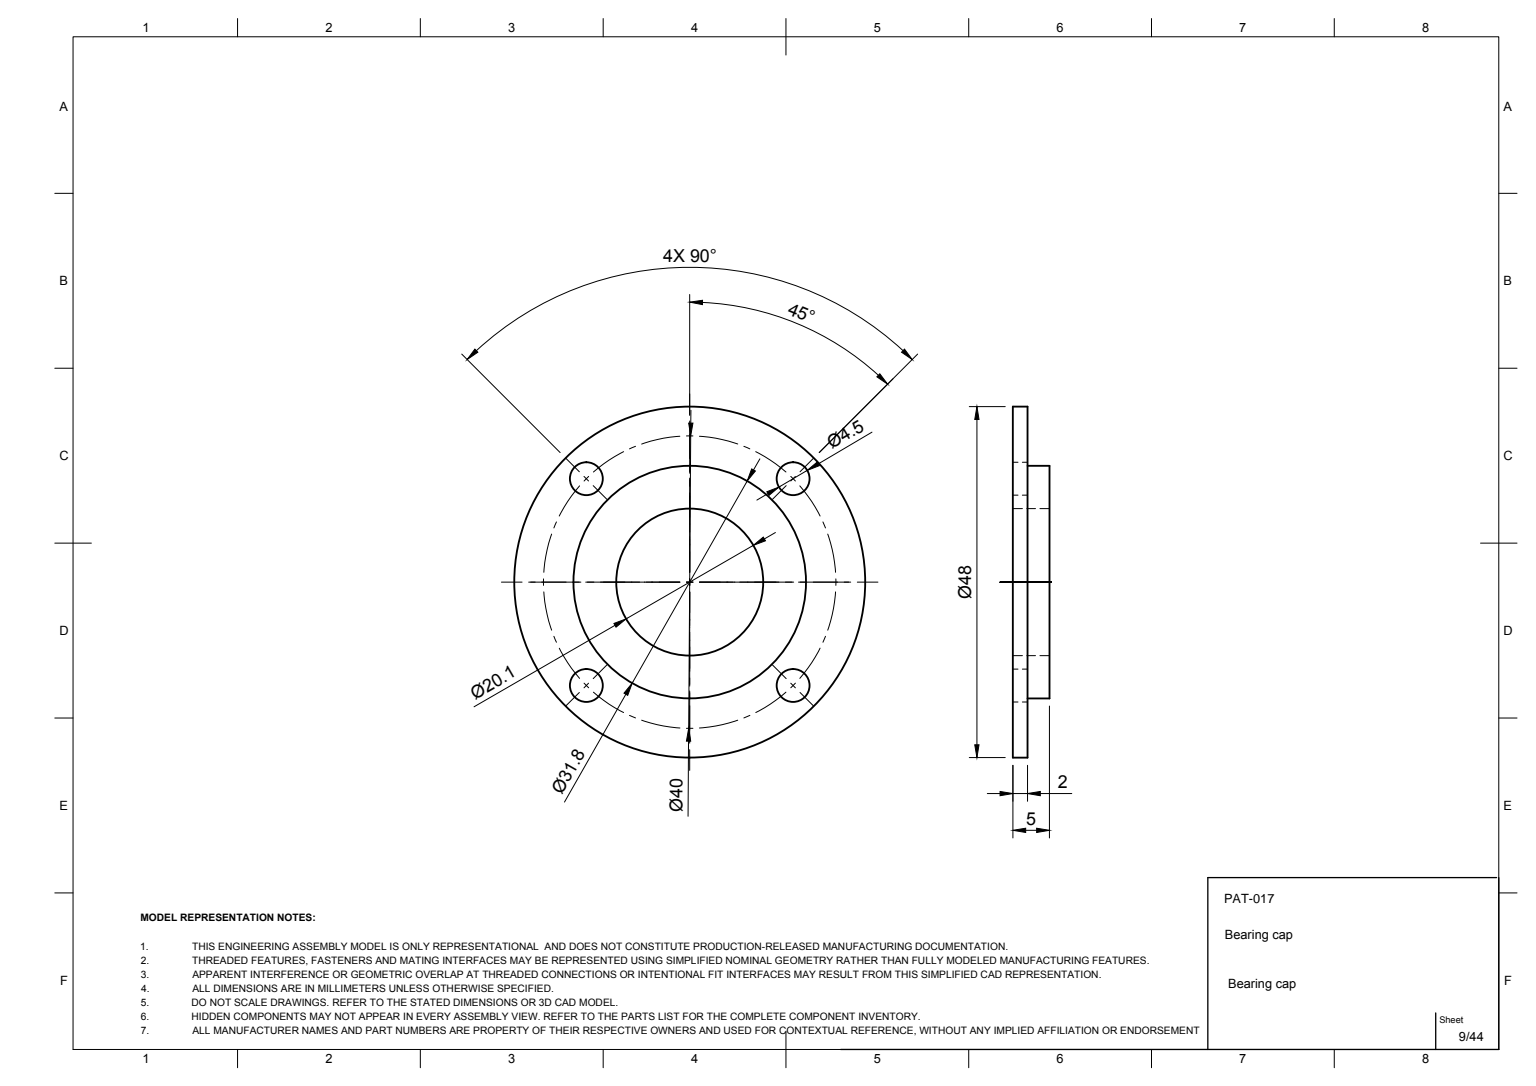
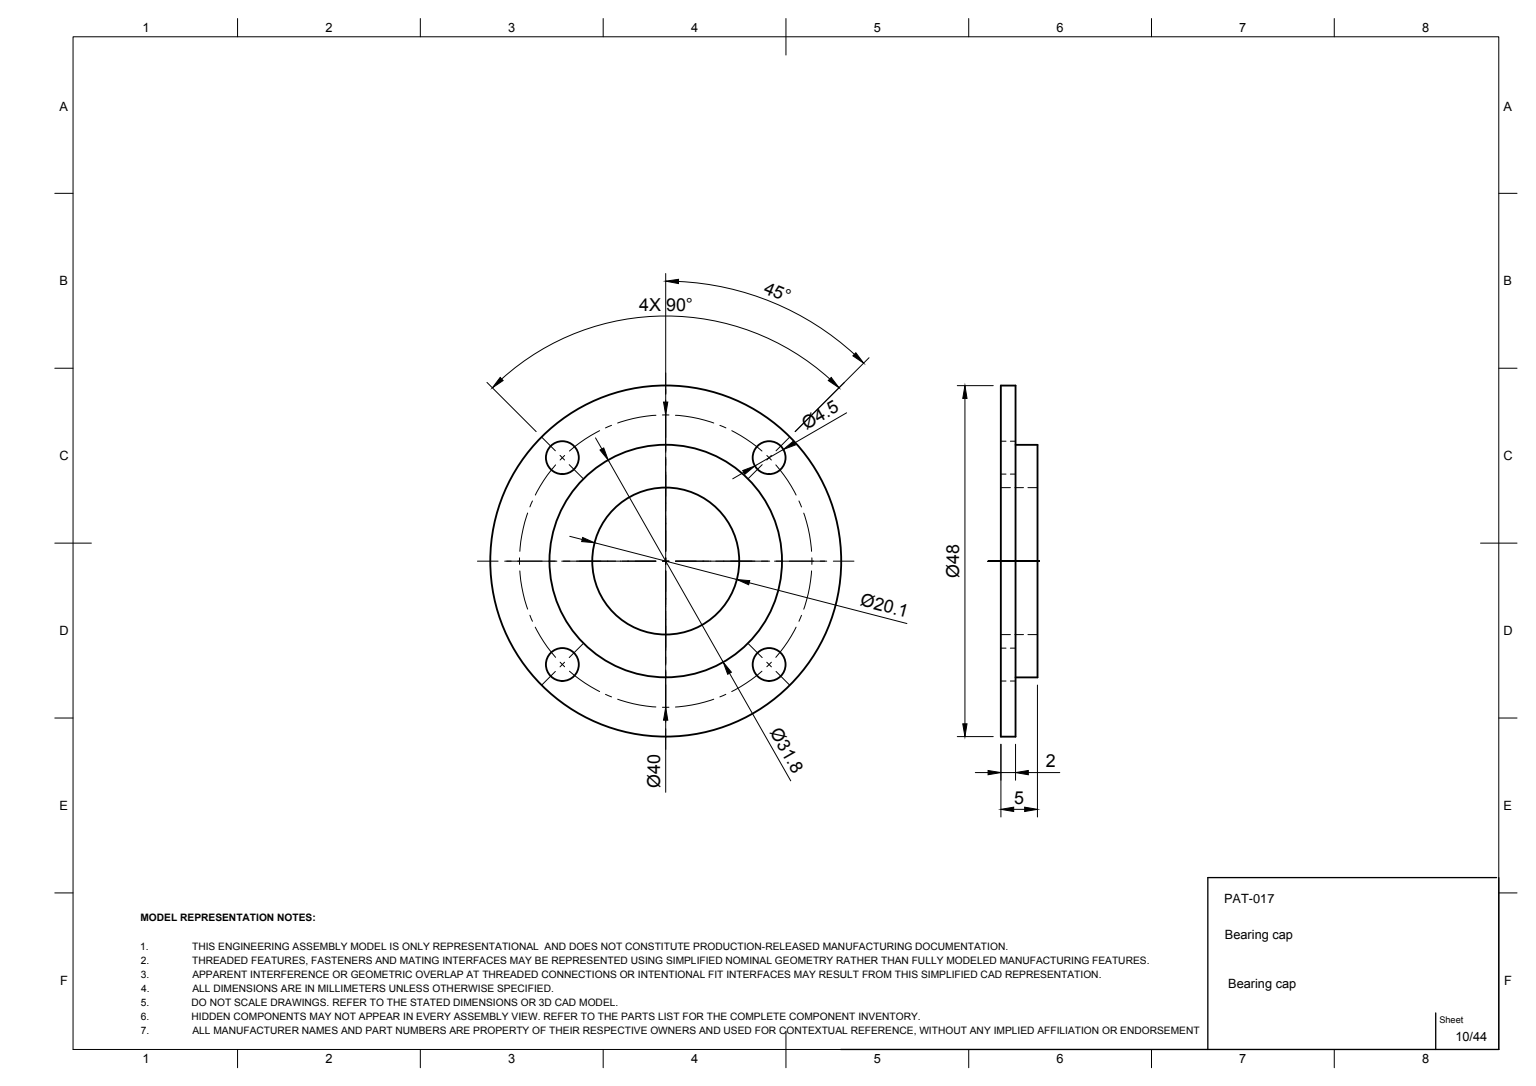
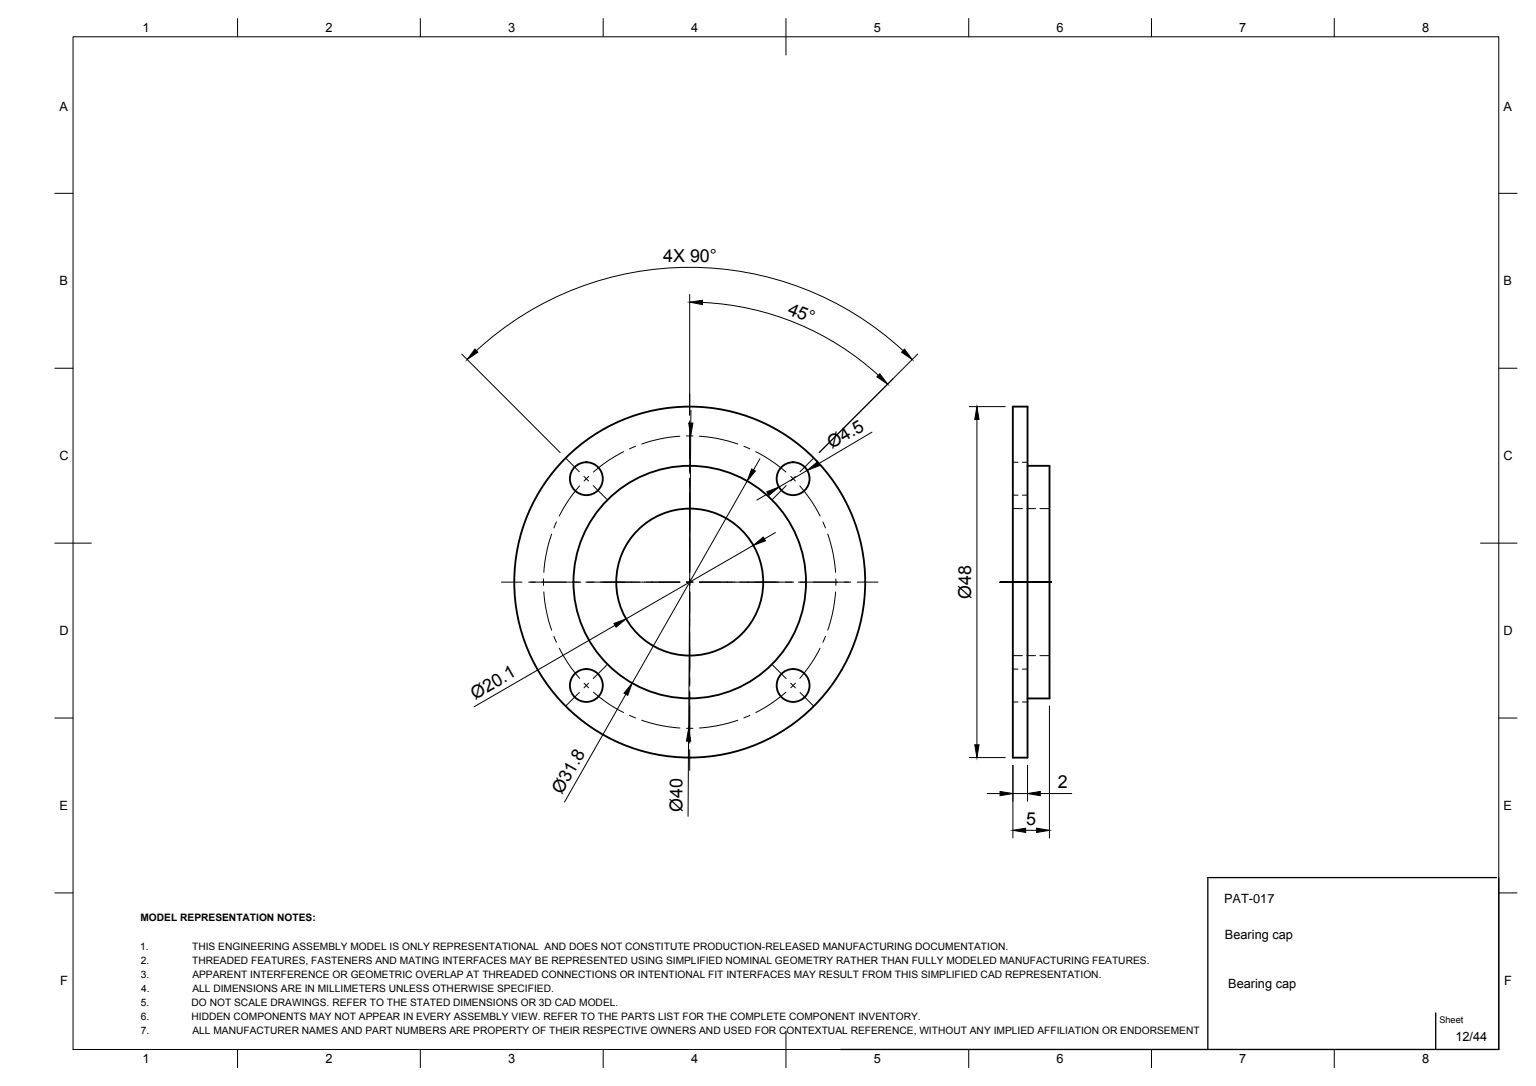
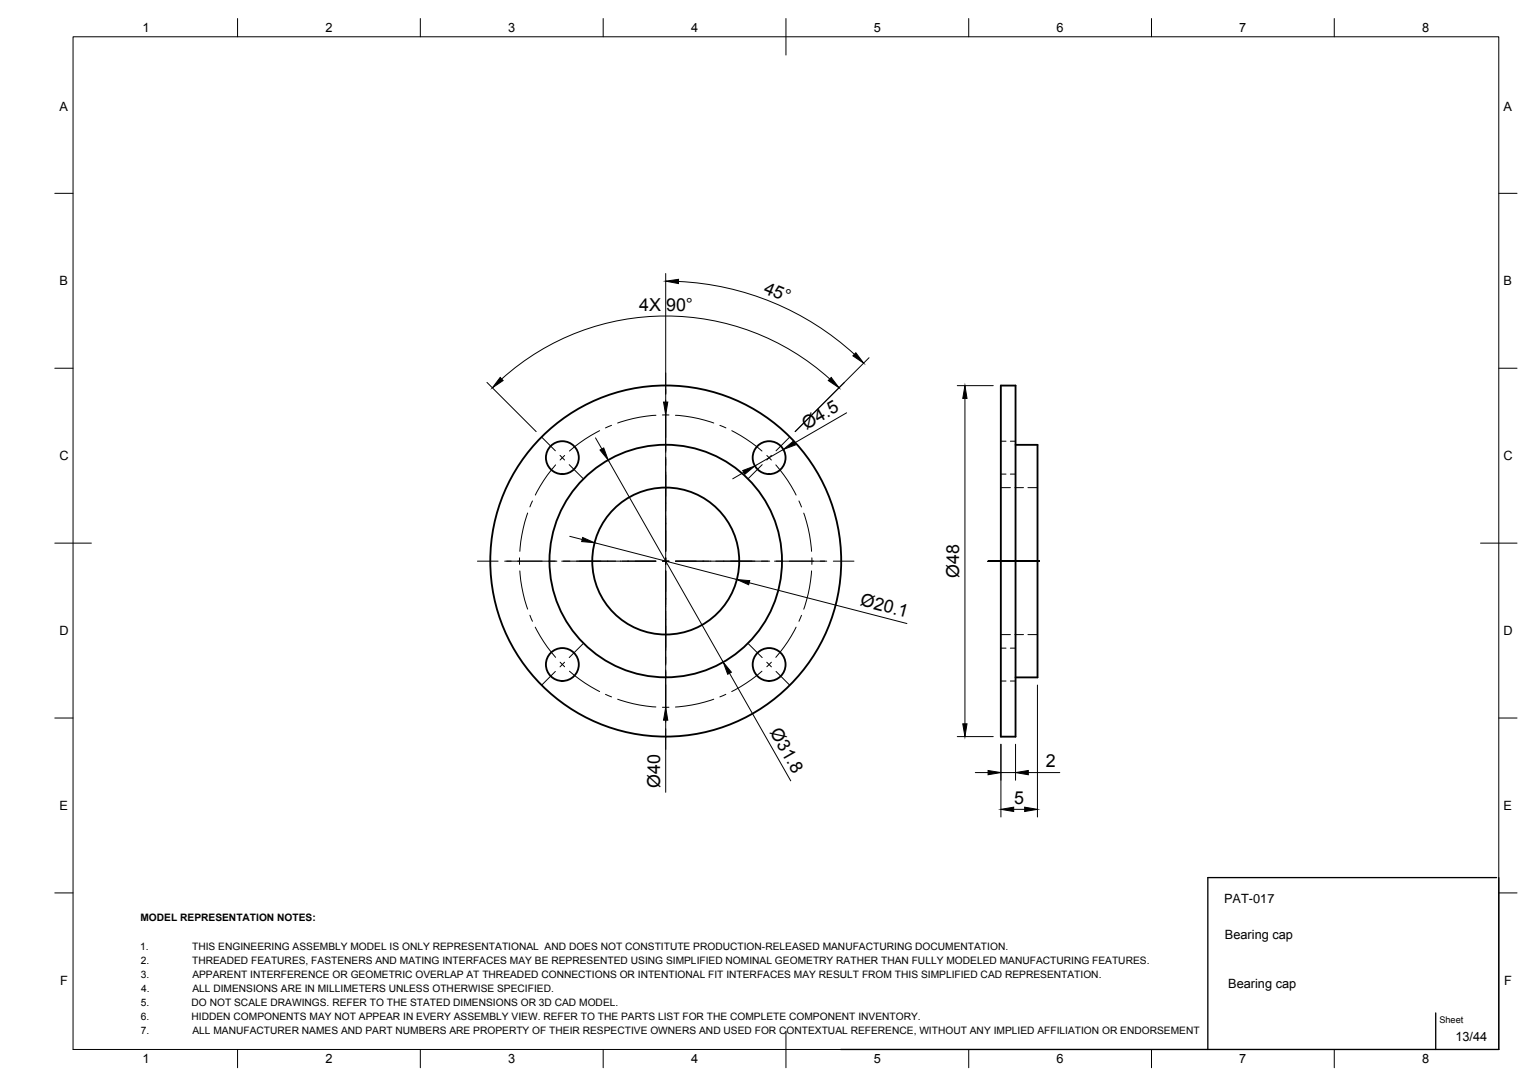
ISO-10303-21;
HEADER;
/* Generated by software containing ST-Developer
 * from STEP Tools, Inc. (www.steptools.com) 
 */

FILE_DESCRIPTION(
/* description */ ('Cam-and-follower valve demonstrator'),
/* implementation_level */ '2;1');

FILE_NAME(
/* name */ 'Bearing cap.step',
/* time_stamp */ '2026-10-28T03:25:17-07:00',
/* author */ (''),
/* organization */ (''),
/* preprocessor_version */ 'ST-DEVELOPER v20.2',
/* originating_system */ 'Autodesk Translation Framework v15.17.0.0',
/* authorisation */ '');

FILE_SCHEMA (('AUTOMOTIVE_DESIGN { 1 0 10303 214 3 1 1 }'));
ENDSEC;

DATA;
#10=MECHANICAL_DESIGN_GEOMETRIC_PRESENTATION_REPRESENTATION('',(#416),#12896);
#344=SHAPE_REPRESENTATION_RELATIONSHIP('SRR','None',#13060,#380);
#380=ADVANCED_BREP_SHAPE_REPRESENTATION('',(#459),#12860);
#416=STYLED_ITEM('',(#13330),#459);
#459=MANIFOLD_SOLID_BREP('Body1',#6183);
#522=FACE_BOUND('',#1542,.T.);
#523=FACE_BOUND('',#1546,.T.);
#524=FACE_BOUND('',#1547,.T.);
#525=FACE_BOUND('',#1548,.T.);
#526=FACE_BOUND('',#1549,.T.);
#527=FACE_BOUND('',#1550,.T.);
#528=FACE_BOUND('',#1552,.T.);
#529=FACE_BOUND('',#1553,.T.);
#530=FACE_BOUND('',#1554,.T.);
#531=FACE_BOUND('',#1555,.T.);
#532=FACE_BOUND('',#1556,.T.);
#685=CIRCLE('',#6702,0.225);
#686=CIRCLE('',#6703,0.225);
#687=CIRCLE('',#6705,0.225);
#688=CIRCLE('',#6706,0.225);
#689=CIRCLE('',#6708,0.225);
#690=CIRCLE('',#6709,0.225);
#691=CIRCLE('',#6711,0.225);
#692=CIRCLE('',#6712,0.225);
#693=CIRCLE('',#6714,1.59);
#694=CIRCLE('',#6715,1.59);
#695=CIRCLE('',#6717,1.005);
#696=CIRCLE('',#6719,1.005);
#697=CIRCLE('',#6721,2.4);
#698=CIRCLE('',#6722,2.4);
#986=CYLINDRICAL_SURFACE('',#6701,0.225);
#987=CYLINDRICAL_SURFACE('',#6704,0.225);
#988=CYLINDRICAL_SURFACE('',#6707,0.225);
#989=CYLINDRICAL_SURFACE('',#6710,0.225);
#990=CYLINDRICAL_SURFACE('',#6713,1.59);
#991=CYLINDRICAL_SURFACE('',#6718,1.005);
#992=CYLINDRICAL_SURFACE('',#6720,2.4);
#1141=FACE_OUTER_BOUND('',#1536,.T.);
#1142=FACE_OUTER_BOUND('',#1537,.T.);
#1143=FACE_OUTER_BOUND('',#1538,.T.);
#1144=FACE_OUTER_BOUND('',#1539,.T.);
#1145=FACE_OUTER_BOUND('',#1540,.T.);
#1146=FACE_OUTER_BOUND('',#1541,.T.);
#1147=FACE_OUTER_BOUND('',#1543,.T.);
#1148=FACE_OUTER_BOUND('',#1544,.T.);
#1149=FACE_OUTER_BOUND('',#1545,.T.);
#1150=FACE_OUTER_BOUND('',#1551,.T.);
#1536=EDGE_LOOP('',(#4317,#4318,#4319,#4320));
#1537=EDGE_LOOP('',(#4321,#4322,#4323,#4324));
#1538=EDGE_LOOP('',(#4325,#4326,#4327,#4328));
#1539=EDGE_LOOP('',(#4329,#4330,#4331,#4332));
#1540=EDGE_LOOP('',(#4333,#4334,#4335,#4336));
#1541=EDGE_LOOP('',(#4337));
#1542=EDGE_LOOP('',(#4338));
#1543=EDGE_LOOP('',(#4339,#4340,#4341,#4342));
#1544=EDGE_LOOP('',(#4343,#4344,#4345,#4346));
#1545=EDGE_LOOP('',(#4347));
#1546=EDGE_LOOP('',(#4348));
#1547=EDGE_LOOP('',(#4349));
#1548=EDGE_LOOP('',(#4350));
#1549=EDGE_LOOP('',(#4351));
#1550=EDGE_LOOP('',(#4352));
#1551=EDGE_LOOP('',(#4353));
#1552=EDGE_LOOP('',(#4354));
#1553=EDGE_LOOP('',(#4355));
#1554=EDGE_LOOP('',(#4356));
#1555=EDGE_LOOP('',(#4357));
#1556=EDGE_LOOP('',(#4358));
#2080=LINE('',#9662,#2502);
#2081=LINE('',#9668,#2503);
#2082=LINE('',#9674,#2504);
#2083=LINE('',#9680,#2505);
#2084=LINE('',#9686,#2506);
#2085=LINE('',#9693,#2507);
#2086=LINE('',#9699,#2508);
#2502=VECTOR('',#7661,0.225);
#2503=VECTOR('',#7668,0.225);
#2504=VECTOR('',#7675,0.225);
#2505=VECTOR('',#7682,0.225);
#2506=VECTOR('',#7689,1.59);
#2507=VECTOR('',#7698,1.005);
#2508=VECTOR('',#7705,2.4);
#2913=VERTEX_POINT('',#9659);
#2914=VERTEX_POINT('',#9661);
#2915=VERTEX_POINT('',#9665);
#2916=VERTEX_POINT('',#9667);
#2917=VERTEX_POINT('',#9671);
#2918=VERTEX_POINT('',#9673);
#2919=VERTEX_POINT('',#9677);
#2920=VERTEX_POINT('',#9679);
#2921=VERTEX_POINT('',#9683);
#2922=VERTEX_POINT('',#9685);
#2923=VERTEX_POINT('',#9689);
#2924=VERTEX_POINT('',#9692);
#2925=VERTEX_POINT('',#9696);
#2926=VERTEX_POINT('',#9698);
#3455=EDGE_CURVE('',#2913,#2913,#685,.T.);
#3456=EDGE_CURVE('',#2913,#2914,#2080,.T.);
#3457=EDGE_CURVE('',#2914,#2914,#686,.T.);
#3458=EDGE_CURVE('',#2915,#2915,#687,.T.);
#3459=EDGE_CURVE('',#2915,#2916,#2081,.T.);
#3460=EDGE_CURVE('',#2916,#2916,#688,.T.);
#3461=EDGE_CURVE('',#2917,#2917,#689,.T.);
#3462=EDGE_CURVE('',#2917,#2918,#2082,.T.);
#3463=EDGE_CURVE('',#2918,#2918,#690,.T.);
#3464=EDGE_CURVE('',#2919,#2919,#691,.T.);
#3465=EDGE_CURVE('',#2919,#2920,#2083,.T.);
#3466=EDGE_CURVE('',#2920,#2920,#692,.T.);
#3467=EDGE_CURVE('',#2921,#2921,#693,.T.);
#3468=EDGE_CURVE('',#2921,#2922,#2084,.T.);
#3469=EDGE_CURVE('',#2922,#2922,#694,.T.);
#3470=EDGE_CURVE('',#2923,#2923,#695,.T.);
#3471=EDGE_CURVE('',#2923,#2924,#2085,.T.);
#3472=EDGE_CURVE('',#2924,#2924,#696,.T.);
#3473=EDGE_CURVE('',#2925,#2925,#697,.T.);
#3474=EDGE_CURVE('',#2925,#2926,#2086,.T.);
#3475=EDGE_CURVE('',#2926,#2926,#698,.T.);
#4317=ORIENTED_EDGE('',*,*,#3455,.F.);
#4318=ORIENTED_EDGE('',*,*,#3456,.T.);
#4319=ORIENTED_EDGE('',*,*,#3457,.F.);
#4320=ORIENTED_EDGE('',*,*,#3456,.F.);
#4321=ORIENTED_EDGE('',*,*,#3458,.F.);
#4322=ORIENTED_EDGE('',*,*,#3459,.T.);
#4323=ORIENTED_EDGE('',*,*,#3460,.F.);
#4324=ORIENTED_EDGE('',*,*,#3459,.F.);
#4325=ORIENTED_EDGE('',*,*,#3461,.F.);
#4326=ORIENTED_EDGE('',*,*,#3462,.T.);
#4327=ORIENTED_EDGE('',*,*,#3463,.F.);
#4328=ORIENTED_EDGE('',*,*,#3462,.F.);
#4329=ORIENTED_EDGE('',*,*,#3464,.F.);
#4330=ORIENTED_EDGE('',*,*,#3465,.T.);
#4331=ORIENTED_EDGE('',*,*,#3466,.F.);
#4332=ORIENTED_EDGE('',*,*,#3465,.F.);
#4333=ORIENTED_EDGE('',*,*,#3467,.F.);
#4334=ORIENTED_EDGE('',*,*,#3468,.T.);
#4335=ORIENTED_EDGE('',*,*,#3469,.F.);
#4336=ORIENTED_EDGE('',*,*,#3468,.F.);
#4337=ORIENTED_EDGE('',*,*,#3467,.T.);
#4338=ORIENTED_EDGE('',*,*,#3470,.T.);
#4339=ORIENTED_EDGE('',*,*,#3470,.F.);
#4340=ORIENTED_EDGE('',*,*,#3471,.T.);
#4341=ORIENTED_EDGE('',*,*,#3472,.T.);
#4342=ORIENTED_EDGE('',*,*,#3471,.F.);
#4343=ORIENTED_EDGE('',*,*,#3473,.F.);
#4344=ORIENTED_EDGE('',*,*,#3474,.T.);
#4345=ORIENTED_EDGE('',*,*,#3475,.T.);
#4346=ORIENTED_EDGE('',*,*,#3474,.F.);
#4347=ORIENTED_EDGE('',*,*,#3473,.T.);
#4348=ORIENTED_EDGE('',*,*,#3469,.T.);
#4349=ORIENTED_EDGE('',*,*,#3466,.T.);
#4350=ORIENTED_EDGE('',*,*,#3463,.T.);
#4351=ORIENTED_EDGE('',*,*,#3460,.T.);
#4352=ORIENTED_EDGE('',*,*,#3457,.T.);
#4353=ORIENTED_EDGE('',*,*,#3475,.F.);
#4354=ORIENTED_EDGE('',*,*,#3472,.F.);
#4355=ORIENTED_EDGE('',*,*,#3464,.T.);
#4356=ORIENTED_EDGE('',*,*,#3461,.T.);
#4357=ORIENTED_EDGE('',*,*,#3458,.T.);
#4358=ORIENTED_EDGE('',*,*,#3455,.T.);
#5630=PLANE('',#6716);
#5631=PLANE('',#6723);
#5632=PLANE('',#6724);
#5857=ADVANCED_FACE('',(#1141),#986,.F.);
#5858=ADVANCED_FACE('',(#1142),#987,.F.);
#5859=ADVANCED_FACE('',(#1143),#988,.F.);
#5860=ADVANCED_FACE('',(#1144),#989,.F.);
#5861=ADVANCED_FACE('',(#1145),#990,.T.);
#5862=ADVANCED_FACE('',(#1146,#522),#5630,.T.);
#5863=ADVANCED_FACE('',(#1147),#991,.F.);
#5864=ADVANCED_FACE('',(#1148),#992,.T.);
#5865=ADVANCED_FACE('',(#1149,#523,#524,#525,#526,#527),#5631,.T.);
#5866=ADVANCED_FACE('',(#1150,#528,#529,#530,#531,#532),#5632,.F.);
#6183=CLOSED_SHELL('',(#5857,#5858,#5859,#5860,#5861,#5862,#5863,#5864,
#5865,#5866));
#6700=AXIS2_PLACEMENT_3D('',#9657,#7655,#7656);
#6701=AXIS2_PLACEMENT_3D('',#9658,#7657,#7658);
#6702=AXIS2_PLACEMENT_3D('',#9660,#7659,#7660);
#6703=AXIS2_PLACEMENT_3D('',#9663,#7662,#7663);
#6704=AXIS2_PLACEMENT_3D('',#9664,#7664,#7665);
#6705=AXIS2_PLACEMENT_3D('',#9666,#7666,#7667);
#6706=AXIS2_PLACEMENT_3D('',#9669,#7669,#7670);
#6707=AXIS2_PLACEMENT_3D('',#9670,#7671,#7672);
#6708=AXIS2_PLACEMENT_3D('',#9672,#7673,#7674);
#6709=AXIS2_PLACEMENT_3D('',#9675,#7676,#7677);
#6710=AXIS2_PLACEMENT_3D('',#9676,#7678,#7679);
#6711=AXIS2_PLACEMENT_3D('',#9678,#7680,#7681);
#6712=AXIS2_PLACEMENT_3D('',#9681,#7683,#7684);
#6713=AXIS2_PLACEMENT_3D('',#9682,#7685,#7686);
#6714=AXIS2_PLACEMENT_3D('',#9684,#7687,#7688);
#6715=AXIS2_PLACEMENT_3D('',#9687,#7690,#7691);
#6716=AXIS2_PLACEMENT_3D('',#9688,#7692,#7693);
#6717=AXIS2_PLACEMENT_3D('',#9690,#7694,#7695);
#6718=AXIS2_PLACEMENT_3D('',#9691,#7696,#7697);
#6719=AXIS2_PLACEMENT_3D('',#9694,#7699,#7700);
#6720=AXIS2_PLACEMENT_3D('',#9695,#7701,#7702);
#6721=AXIS2_PLACEMENT_3D('',#9697,#7703,#7704);
#6722=AXIS2_PLACEMENT_3D('',#9700,#7706,#7707);
#6723=AXIS2_PLACEMENT_3D('',#9701,#7708,#7709);
#6724=AXIS2_PLACEMENT_3D('',#9702,#7710,#7711);
#7655=DIRECTION('axis',(0.,0.,1.));
#7656=DIRECTION('refdir',(1.,0.,0.));
#7657=DIRECTION('center_axis',(0.,1.,0.));
#7658=DIRECTION('ref_axis',(1.,0.,0.));
#7659=DIRECTION('center_axis',(0.,1.,0.));
#7660=DIRECTION('ref_axis',(1.,0.,0.));
#7661=DIRECTION('',(0.,1.,0.));
#7662=DIRECTION('center_axis',(0.,-1.,0.));
#7663=DIRECTION('ref_axis',(1.,0.,0.));
#7664=DIRECTION('center_axis',(0.,1.,0.));
#7665=DIRECTION('ref_axis',(1.,0.,0.));
#7666=DIRECTION('center_axis',(0.,1.,0.));
#7667=DIRECTION('ref_axis',(1.,0.,0.));
#7668=DIRECTION('',(0.,1.,0.));
#7669=DIRECTION('center_axis',(0.,-1.,0.));
#7670=DIRECTION('ref_axis',(1.,0.,0.));
#7671=DIRECTION('center_axis',(0.,1.,0.));
#7672=DIRECTION('ref_axis',(1.,0.,0.));
#7673=DIRECTION('center_axis',(0.,1.,0.));
#7674=DIRECTION('ref_axis',(1.,0.,0.));
#7675=DIRECTION('',(0.,1.,0.));
#7676=DIRECTION('center_axis',(0.,-1.,0.));
#7677=DIRECTION('ref_axis',(1.,0.,0.));
#7678=DIRECTION('center_axis',(0.,1.,0.));
#7679=DIRECTION('ref_axis',(1.,0.,0.));
#7680=DIRECTION('center_axis',(0.,1.,0.));
#7681=DIRECTION('ref_axis',(1.,0.,0.));
#7682=DIRECTION('',(0.,1.,0.));
#7683=DIRECTION('center_axis',(0.,-1.,0.));
#7684=DIRECTION('ref_axis',(1.,0.,0.));
#7685=DIRECTION('center_axis',(0.,1.,0.));
#7686=DIRECTION('ref_axis',(1.,0.,0.));
#7687=DIRECTION('center_axis',(0.,1.,0.));
#7688=DIRECTION('ref_axis',(1.,0.,0.));
#7689=DIRECTION('',(0.,-1.,0.));
#7690=DIRECTION('center_axis',(0.,-1.,0.));
#7691=DIRECTION('ref_axis',(1.,0.,0.));
#7692=DIRECTION('center_axis',(0.,1.,0.));
#7693=DIRECTION('ref_axis',(1.,0.,0.));
#7694=DIRECTION('center_axis',(0.,-1.,0.));
#7695=DIRECTION('ref_axis',(1.,0.,0.));
#7696=DIRECTION('center_axis',(0.,1.,0.));
#7697=DIRECTION('ref_axis',(1.,0.,0.));
#7698=DIRECTION('',(0.,-1.,0.));
#7699=DIRECTION('center_axis',(0.,-1.,0.));
#7700=DIRECTION('ref_axis',(1.,0.,0.));
#7701=DIRECTION('center_axis',(0.,1.,0.));
#7702=DIRECTION('ref_axis',(1.,0.,0.));
#7703=DIRECTION('center_axis',(0.,1.,0.));
#7704=DIRECTION('ref_axis',(1.,0.,0.));
#7705=DIRECTION('',(0.,-1.,0.));
#7706=DIRECTION('center_axis',(0.,1.,0.));
#7707=DIRECTION('ref_axis',(1.,0.,0.));
#7708=DIRECTION('center_axis',(0.,1.,0.));
#7709=DIRECTION('ref_axis',(1.,0.,0.));
#7710=DIRECTION('center_axis',(0.,1.,0.));
#7711=DIRECTION('ref_axis',(1.,0.,0.));
#9657=CARTESIAN_POINT('',(0.,0.,0.));
#9658=CARTESIAN_POINT('Origin',(-1.4142135623731,-3.6,2.58578643762691));
#9659=CARTESIAN_POINT('',(-1.6392135623731,-3.5,2.58578643762691));
#9660=CARTESIAN_POINT('Origin',(-1.4142135623731,-3.5,2.58578643762691));
#9661=CARTESIAN_POINT('',(-1.6392135623731,-3.3,2.58578643762691));
#9662=CARTESIAN_POINT('',(-1.6392135623731,-3.6,2.58578643762691));
#9663=CARTESIAN_POINT('Origin',(-1.4142135623731,-3.3,2.58578643762691));
#9664=CARTESIAN_POINT('Origin',(-1.41421356237309,-3.6,5.41421356237309));
#9665=CARTESIAN_POINT('',(-1.6392135623731,-3.5,5.41421356237309));
#9666=CARTESIAN_POINT('Origin',(-1.41421356237309,-3.5,5.41421356237309));
#9667=CARTESIAN_POINT('',(-1.6392135623731,-3.3,5.41421356237309));
#9668=CARTESIAN_POINT('',(-1.6392135623731,-3.6,5.41421356237309));
#9669=CARTESIAN_POINT('Origin',(-1.41421356237309,-3.3,5.41421356237309));
#9670=CARTESIAN_POINT('Origin',(1.4142135623731,-3.6,5.41421356237309));
#9671=CARTESIAN_POINT('',(1.1892135623731,-3.5,5.41421356237309));
#9672=CARTESIAN_POINT('Origin',(1.4142135623731,-3.5,5.41421356237309));
#9673=CARTESIAN_POINT('',(1.1892135623731,-3.3,5.41421356237309));
#9674=CARTESIAN_POINT('',(1.1892135623731,-3.6,5.41421356237309));
#9675=CARTESIAN_POINT('Origin',(1.4142135623731,-3.3,5.41421356237309));
#9676=CARTESIAN_POINT('Origin',(1.41421356237309,-3.6,2.5857864376269));
#9677=CARTESIAN_POINT('',(1.18921356237309,-3.5,2.5857864376269));
#9678=CARTESIAN_POINT('Origin',(1.41421356237309,-3.5,2.5857864376269));
#9679=CARTESIAN_POINT('',(1.18921356237309,-3.3,2.5857864376269));
#9680=CARTESIAN_POINT('',(1.18921356237309,-3.6,2.5857864376269));
#9681=CARTESIAN_POINT('Origin',(1.41421356237309,-3.3,2.5857864376269));
#9682=CARTESIAN_POINT('Origin',(0.,-3.3,4.));
#9683=CARTESIAN_POINT('',(-1.59,-3.,4.));
#9684=CARTESIAN_POINT('Origin',(0.,-3.,4.));
#9685=CARTESIAN_POINT('',(-1.59,-3.3,4.));
#9686=CARTESIAN_POINT('',(-1.59,-3.3,4.));
#9687=CARTESIAN_POINT('Origin',(0.,-3.3,4.));
#9688=CARTESIAN_POINT('Origin',(0.,-3.,4.));
#9689=CARTESIAN_POINT('',(-1.005,-3.,4.));
#9690=CARTESIAN_POINT('Origin',(0.,-3.,4.));
#9691=CARTESIAN_POINT('Origin',(0.,-3.5,4.));
#9692=CARTESIAN_POINT('',(-1.005,-3.5,4.));
#9693=CARTESIAN_POINT('',(-1.005,-3.5,4.));
#9694=CARTESIAN_POINT('Origin',(0.,-3.5,4.));
#9695=CARTESIAN_POINT('Origin',(0.,-3.5,4.));
#9696=CARTESIAN_POINT('',(-2.4,-3.3,4.));
#9697=CARTESIAN_POINT('Origin',(0.,-3.3,4.));
#9698=CARTESIAN_POINT('',(-2.4,-3.5,4.));
#9699=CARTESIAN_POINT('',(-2.4,-3.5,4.));
#9700=CARTESIAN_POINT('Origin',(0.,-3.5,4.));
#9701=CARTESIAN_POINT('Origin',(0.,-3.3,4.));
#9702=CARTESIAN_POINT('Origin',(0.,-3.5,4.));
#12817=UNCERTAINTY_MEASURE_WITH_UNIT(LENGTH_MEASURE(0.001),#12897,
'DISTANCE_ACCURACY_VALUE',
'Maximum model space distance between geometric entities at asserted c
onnectivities');
#12853=UNCERTAINTY_MEASURE_WITH_UNIT(LENGTH_MEASURE(0.001),#12897,
'DISTANCE_ACCURACY_VALUE',
'Maximum model space distance between geometric entities at asserted c
onnectivities');
#12860=(
GEOMETRIC_REPRESENTATION_CONTEXT(3)
GLOBAL_UNCERTAINTY_ASSIGNED_CONTEXT((#12817))
GLOBAL_UNIT_ASSIGNED_CONTEXT((#12897,#12899,#12900))
REPRESENTATION_CONTEXT('','3D')
);
#12896=(
GEOMETRIC_REPRESENTATION_CONTEXT(3)
GLOBAL_UNCERTAINTY_ASSIGNED_CONTEXT((#12853))
GLOBAL_UNIT_ASSIGNED_CONTEXT((#12897,#12899,#12900))
REPRESENTATION_CONTEXT('','3D')
);
#12897=(
LENGTH_UNIT()
NAMED_UNIT(*)
SI_UNIT(.CENTI.,.METRE.)
);
#12899=(
NAMED_UNIT(*)
PLANE_ANGLE_UNIT()
SI_UNIT($,.RADIAN.)
);
#12900=(
NAMED_UNIT(*)
SI_UNIT($,.STERADIAN.)
SOLID_ANGLE_UNIT()
);
#12907=SHAPE_DEFINITION_REPRESENTATION(#12949,#13060);
#12949=PRODUCT_DEFINITION_SHAPE('',$,#13103);
#13060=SHAPE_REPRESENTATION('',(#6700),#12860);
#13096=PRODUCT_DEFINITION_CONTEXT('part definition',#13224,'design');
#13103=PRODUCT_DEFINITION('Bearing cap','Bearing cap',#13145,#13096);
#13145=PRODUCT_DEFINITION_FORMATION('',$,#13232);
#13224=APPLICATION_CONTEXT(
'Core Data for Automotive Mechanical Design Process');
#13225=PRODUCT_CONTEXT('part definition',#13224,'mechanical');
#13232=PRODUCT('Bearing cap','Bearing cap','Bearing cap',(#13225));
#13324=COLOUR_RGB('Grey',0.48,0.52,0.57);
#13325=FILL_AREA_STYLE_COLOUR('',#13324);
#13326=FILL_AREA_STYLE('',(#13325));
#13327=SURFACE_STYLE_FILL_AREA(#13326);
#13328=SURFACE_SIDE_STYLE('',(#13327));
#13329=SURFACE_STYLE_USAGE(.BOTH.,#13328);
#13330=PRESENTATION_STYLE_ASSIGNMENT((#13329));
ENDSEC;
END-ISO-10303-21;
